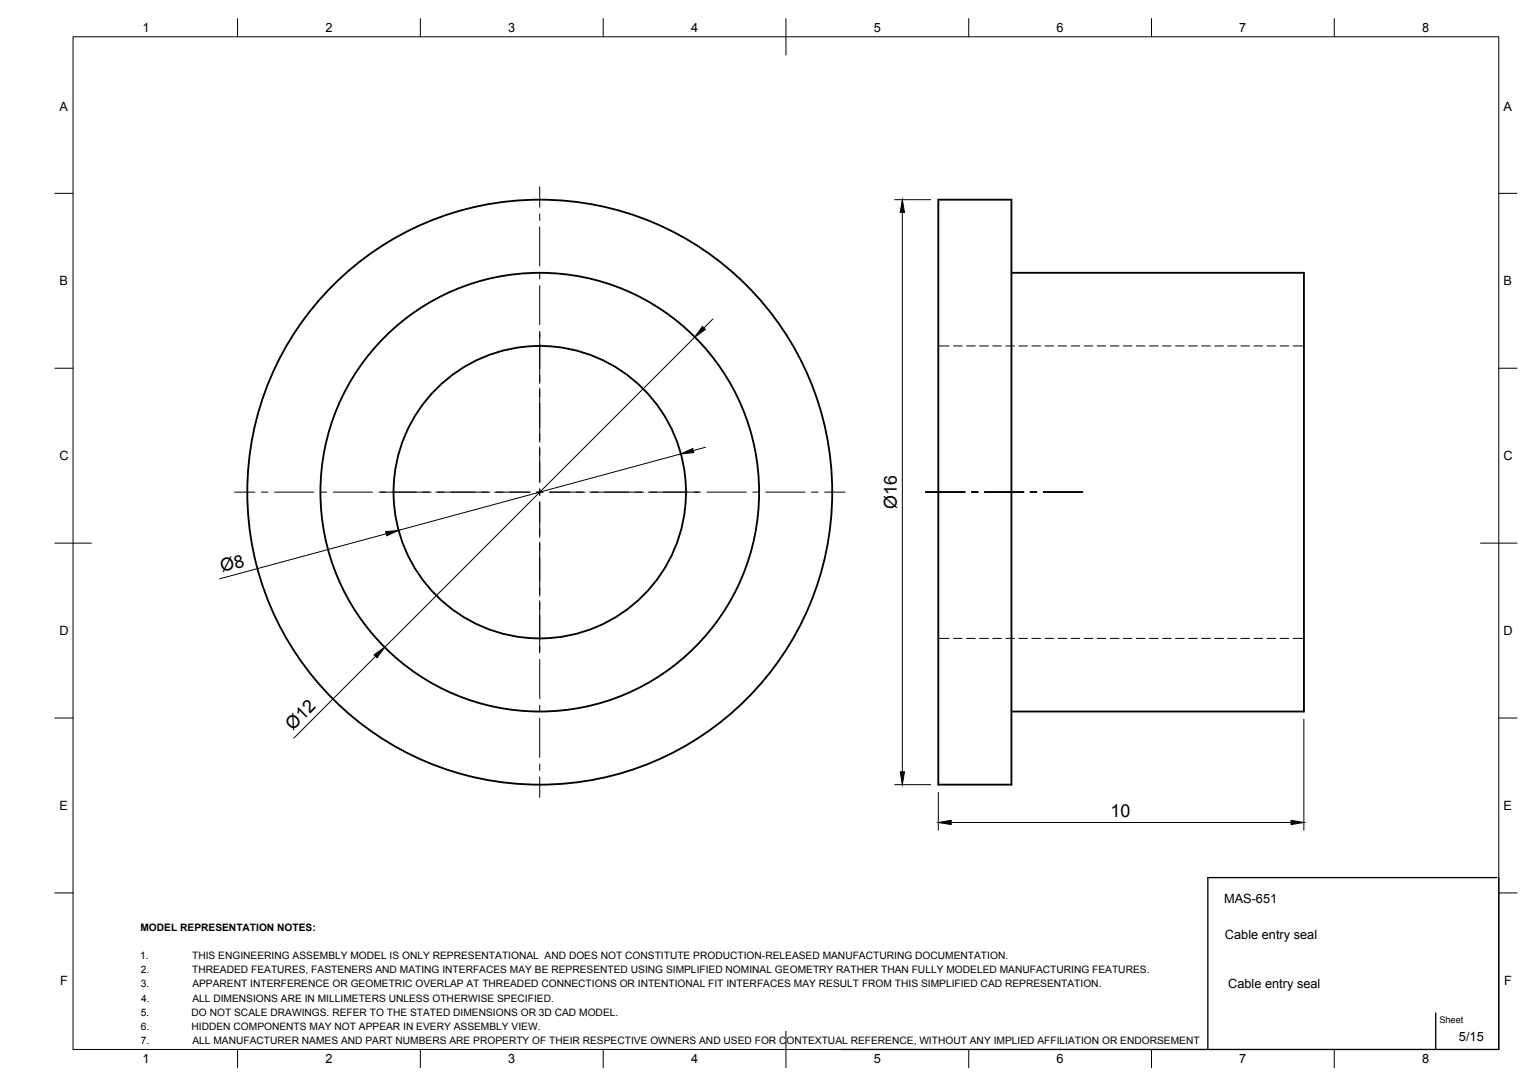
ISO-10303-21;
HEADER;
/* Generated by software containing ST-Developer
 * from STEP Tools, Inc. (www.steptools.com) 
 */

FILE_DESCRIPTION(
/* description */ ('Independent direct-acting normally-closed roller-plunger limit-switch
 CAD. Removable cover, insulated terminal supports, captured bus/conta
ct bridge, native Coil return spring, integral lower travel stop, reus
able instanced hardware and free roller. Manual geometric contact open
ing4mm; no snap-action/contact-force, electrical/current/voltage, envi
ronmental seal, safety-switch, wear, load or life certification. Exter
nal wiring and anchors omitted; fits and application engineering requi
red.'),
/* implementation_level */ '2;1');

FILE_NAME(
/* name */ 'Cable entry seal.step',
/* time_stamp */ '2026-11-08T07:32:43-08:00',
/* author */ (''),
/* organization */ (''),
/* preprocessor_version */ 'ST-DEVELOPER v20.2',
/* originating_system */ 'Autodesk Translation Framework v15.17.0.0',
/* authorisation */ '');

FILE_SCHEMA (('AUTOMOTIVE_DESIGN { 1 0 10303 214 3 1 1 }'));
ENDSEC;

DATA;
#10=MECHANICAL_DESIGN_GEOMETRIC_PRESENTATION_REPRESENTATION('',(#178),#36482);
#144=SHAPE_REPRESENTATION_RELATIONSHIP('SRR','None',#36557,#161);
#161=ADVANCED_BREP_SHAPE_REPRESENTATION('',(#195),#36467);
#178=STYLED_ITEM('',(#36651),#195);
#195=MANIFOLD_SOLID_BREP('Body1',#9769);
#264=FACE_BOUND('',#1178,.T.);
#265=FACE_BOUND('',#1181,.T.);
#266=FACE_BOUND('',#1185,.T.);
#339=PLANE('',#10195);
#340=PLANE('',#10200);
#341=PLANE('',#10206);
#610=FACE_OUTER_BOUND('',#1177,.T.);
#611=FACE_OUTER_BOUND('',#1179,.T.);
#612=FACE_OUTER_BOUND('',#1180,.T.);
#613=FACE_OUTER_BOUND('',#1182,.T.);
#614=FACE_OUTER_BOUND('',#1183,.T.);
#615=FACE_OUTER_BOUND('',#1184,.T.);
#1177=EDGE_LOOP('',(#6934));
#1178=EDGE_LOOP('',(#6935));
#1179=EDGE_LOOP('',(#6936,#6937,#6938,#6939));
#1180=EDGE_LOOP('',(#6940));
#1181=EDGE_LOOP('',(#6941));
#1182=EDGE_LOOP('',(#6942,#6943,#6944,#6945));
#1183=EDGE_LOOP('',(#6946,#6947,#6948,#6949));
#1184=EDGE_LOOP('',(#6950));
#1185=EDGE_LOOP('',(#6951));
#1638=CIRCLE('',#10196,0.8);
#1639=CIRCLE('',#10197,0.6);
#1640=CIRCLE('',#10199,0.8);
#1641=CIRCLE('',#10201,0.4);
#1642=CIRCLE('',#10203,0.4);
#1643=CIRCLE('',#10205,0.6);
#2627=LINE('',#20464,#3201);
#2628=LINE('',#20472,#3202);
#2629=LINE('',#20476,#3203);
#3201=VECTOR('',#11326,0.8);
#3202=VECTOR('',#11337,0.4);
#3203=VECTOR('',#11342,0.6);
#3909=VERTEX_POINT('',#20458);
#3910=VERTEX_POINT('',#20460);
#3911=VERTEX_POINT('',#20463);
#3912=VERTEX_POINT('',#20467);
#3913=VERTEX_POINT('',#20470);
#3914=VERTEX_POINT('',#20474);
#5023=EDGE_CURVE('',#3909,#3909,#1638,.T.);
#5024=EDGE_CURVE('',#3910,#3910,#1639,.T.);
#5025=EDGE_CURVE('',#3909,#3911,#2627,.T.);
#5026=EDGE_CURVE('',#3911,#3911,#1640,.T.);
#5027=EDGE_CURVE('',#3912,#3912,#1641,.T.);
#5028=EDGE_CURVE('',#3913,#3913,#1642,.T.);
#5029=EDGE_CURVE('',#3913,#3912,#2628,.T.);
#5030=EDGE_CURVE('',#3914,#3914,#1643,.T.);
#5031=EDGE_CURVE('',#3914,#3910,#2629,.T.);
#6934=ORIENTED_EDGE('',*,*,#5023,.T.);
#6935=ORIENTED_EDGE('',*,*,#5024,.F.);
#6936=ORIENTED_EDGE('',*,*,#5023,.F.);
#6937=ORIENTED_EDGE('',*,*,#5025,.T.);
#6938=ORIENTED_EDGE('',*,*,#5026,.T.);
#6939=ORIENTED_EDGE('',*,*,#5025,.F.);
#6940=ORIENTED_EDGE('',*,*,#5026,.F.);
#6941=ORIENTED_EDGE('',*,*,#5027,.F.);
#6942=ORIENTED_EDGE('',*,*,#5028,.F.);
#6943=ORIENTED_EDGE('',*,*,#5029,.T.);
#6944=ORIENTED_EDGE('',*,*,#5027,.T.);
#6945=ORIENTED_EDGE('',*,*,#5029,.F.);
#6946=ORIENTED_EDGE('',*,*,#5030,.F.);
#6947=ORIENTED_EDGE('',*,*,#5031,.T.);
#6948=ORIENTED_EDGE('',*,*,#5024,.T.);
#6949=ORIENTED_EDGE('',*,*,#5031,.F.);
#6950=ORIENTED_EDGE('',*,*,#5030,.T.);
#6951=ORIENTED_EDGE('',*,*,#5028,.T.);
#8986=CYLINDRICAL_SURFACE('',#10198,0.8);
#8987=CYLINDRICAL_SURFACE('',#10202,0.4);
#8988=CYLINDRICAL_SURFACE('',#10204,0.6);
#9400=ADVANCED_FACE('',(#610,#264),#339,.T.);
#9401=ADVANCED_FACE('',(#611),#8986,.T.);
#9402=ADVANCED_FACE('',(#612,#265),#340,.F.);
#9403=ADVANCED_FACE('',(#613),#8987,.F.);
#9404=ADVANCED_FACE('',(#614),#8988,.T.);
#9405=ADVANCED_FACE('',(#615,#266),#341,.T.);
#9769=CLOSED_SHELL('',(#9400,#9401,#9402,#9403,#9404,#9405));
#10194=AXIS2_PLACEMENT_3D('',#20456,#11316,#11317);
#10195=AXIS2_PLACEMENT_3D('',#20457,#11318,#11319);
#10196=AXIS2_PLACEMENT_3D('',#20459,#11320,#11321);
#10197=AXIS2_PLACEMENT_3D('',#20461,#11322,#11323);
#10198=AXIS2_PLACEMENT_3D('',#20462,#11324,#11325);
#10199=AXIS2_PLACEMENT_3D('',#20465,#11327,#11328);
#10200=AXIS2_PLACEMENT_3D('',#20466,#11329,#11330);
#10201=AXIS2_PLACEMENT_3D('',#20468,#11331,#11332);
#10202=AXIS2_PLACEMENT_3D('',#20469,#11333,#11334);
#10203=AXIS2_PLACEMENT_3D('',#20471,#11335,#11336);
#10204=AXIS2_PLACEMENT_3D('',#20473,#11338,#11339);
#10205=AXIS2_PLACEMENT_3D('',#20475,#11340,#11341);
#10206=AXIS2_PLACEMENT_3D('',#20477,#11343,#11344);
#11316=DIRECTION('axis',(0.,0.,1.));
#11317=DIRECTION('refdir',(1.,0.,0.));
#11318=DIRECTION('center_axis',(0.,0.,1.));
#11319=DIRECTION('ref_axis',(1.,0.,0.));
#11320=DIRECTION('center_axis',(0.,0.,1.));
#11321=DIRECTION('ref_axis',(1.,0.,0.));
#11322=DIRECTION('center_axis',(0.,0.,1.));
#11323=DIRECTION('ref_axis',(1.,0.,0.));
#11324=DIRECTION('center_axis',(0.,0.,1.));
#11325=DIRECTION('ref_axis',(1.,0.,0.));
#11326=DIRECTION('',(0.,0.,-1.));
#11327=DIRECTION('center_axis',(0.,0.,1.));
#11328=DIRECTION('ref_axis',(1.,0.,0.));
#11329=DIRECTION('center_axis',(0.,0.,1.));
#11330=DIRECTION('ref_axis',(1.,0.,0.));
#11331=DIRECTION('center_axis',(0.,0.,-1.));
#11332=DIRECTION('ref_axis',(1.,0.,0.));
#11333=DIRECTION('center_axis',(0.,0.,1.));
#11334=DIRECTION('ref_axis',(1.,0.,0.));
#11335=DIRECTION('center_axis',(0.,0.,-1.));
#11336=DIRECTION('ref_axis',(1.,0.,0.));
#11337=DIRECTION('',(0.,0.,-1.));
#11338=DIRECTION('center_axis',(0.,0.,1.));
#11339=DIRECTION('ref_axis',(1.,0.,0.));
#11340=DIRECTION('center_axis',(0.,0.,1.));
#11341=DIRECTION('ref_axis',(1.,0.,0.));
#11342=DIRECTION('',(0.,0.,-1.));
#11343=DIRECTION('center_axis',(0.,0.,1.));
#11344=DIRECTION('ref_axis',(1.,0.,0.));
#20456=CARTESIAN_POINT('',(0.,0.,0.));
#20457=CARTESIAN_POINT('Origin',(0.,0.,0.));
#20458=CARTESIAN_POINT('',(-0.8,-9.79717439317883E-17,0.));
#20459=CARTESIAN_POINT('Origin',(0.,0.,0.));
#20460=CARTESIAN_POINT('',(-0.6,-7.34788079488412E-17,0.));
#20461=CARTESIAN_POINT('Origin',(0.,0.,0.));
#20462=CARTESIAN_POINT('Origin',(0.,0.,-0.2));
#20463=CARTESIAN_POINT('',(-0.8,-9.79717439317883E-17,-0.2));
#20464=CARTESIAN_POINT('',(-0.8,-9.79717439317883E-17,-0.2));
#20465=CARTESIAN_POINT('Origin',(0.,0.,-0.2));
#20466=CARTESIAN_POINT('Origin',(0.,0.,-0.2));
#20467=CARTESIAN_POINT('',(-0.4,-4.89858719658941E-17,-0.2));
#20468=CARTESIAN_POINT('Origin',(0.,0.,-0.2));
#20469=CARTESIAN_POINT('Origin',(0.,0.,0.));
#20470=CARTESIAN_POINT('',(-0.4,-4.89858719658941E-17,0.8));
#20471=CARTESIAN_POINT('Origin',(0.,0.,0.8));
#20472=CARTESIAN_POINT('',(-0.4,-4.89858719658941E-17,0.));
#20473=CARTESIAN_POINT('Origin',(0.,0.,0.));
#20474=CARTESIAN_POINT('',(-0.6,-7.34788079488412E-17,0.8));
#20475=CARTESIAN_POINT('Origin',(0.,0.,0.8));
#20476=CARTESIAN_POINT('',(-0.6,-7.34788079488412E-17,0.));
#20477=CARTESIAN_POINT('Origin',(0.,0.,0.8));
#36448=UNCERTAINTY_MEASURE_WITH_UNIT(LENGTH_MEASURE(0.001),#36483,
'DISTANCE_ACCURACY_VALUE',
'Maximum model space distance between geometric entities at asserted c
onnectivities');
#36463=UNCERTAINTY_MEASURE_WITH_UNIT(LENGTH_MEASURE(0.001),#36483,
'DISTANCE_ACCURACY_VALUE',
'Maximum model space distance between geometric entities at asserted c
onnectivities');
#36467=(
GEOMETRIC_REPRESENTATION_CONTEXT(3)
GLOBAL_UNCERTAINTY_ASSIGNED_CONTEXT((#36448))
GLOBAL_UNIT_ASSIGNED_CONTEXT((#36483,#36485,#36486))
REPRESENTATION_CONTEXT('','3D')
);
#36482=(
GEOMETRIC_REPRESENTATION_CONTEXT(3)
GLOBAL_UNCERTAINTY_ASSIGNED_CONTEXT((#36463))
GLOBAL_UNIT_ASSIGNED_CONTEXT((#36483,#36485,#36486))
REPRESENTATION_CONTEXT('','3D')
);
#36483=(
LENGTH_UNIT()
NAMED_UNIT(*)
SI_UNIT(.CENTI.,.METRE.)
);
#36485=(
NAMED_UNIT(*)
PLANE_ANGLE_UNIT()
SI_UNIT($,.RADIAN.)
);
#36486=(
NAMED_UNIT(*)
SI_UNIT($,.STERADIAN.)
SOLID_ANGLE_UNIT()
);
#36490=SHAPE_DEFINITION_REPRESENTATION(#36508,#36557);
#36508=PRODUCT_DEFINITION_SHAPE('',$,#36576);
#36557=SHAPE_REPRESENTATION('',(#10194),#36467);
#36572=PRODUCT_DEFINITION_CONTEXT('part definition',#36628,'design');
#36576=PRODUCT_DEFINITION('Cable entry seal','Cable entry seal',#36594,
#36572);
#36594=PRODUCT_DEFINITION_FORMATION('',$,#36633);
#36628=APPLICATION_CONTEXT(
'Core Data for Automotive Mechanical Design Process');
#36629=PRODUCT_CONTEXT('part definition',#36628,'mechanical');
#36633=PRODUCT('Cable entry seal','Cable entry seal',$,(#36629));
#36651=PRESENTATION_STYLE_ASSIGNMENT((#36665));
#36665=SURFACE_STYLE_USAGE(.BOTH.,#36679);
#36679=SURFACE_SIDE_STYLE('',(#36693));
#36693=SURFACE_STYLE_FILL_AREA(#36707);
#36707=FILL_AREA_STYLE('Charcoal',(#36721));
#36721=FILL_AREA_STYLE_COLOUR('Charcoal',#36735);
#36735=COLOUR_RGB('Charcoal',0.164705882352941,0.184313725490196,0.211764705882353);
ENDSEC;
END-ISO-10303-21;
